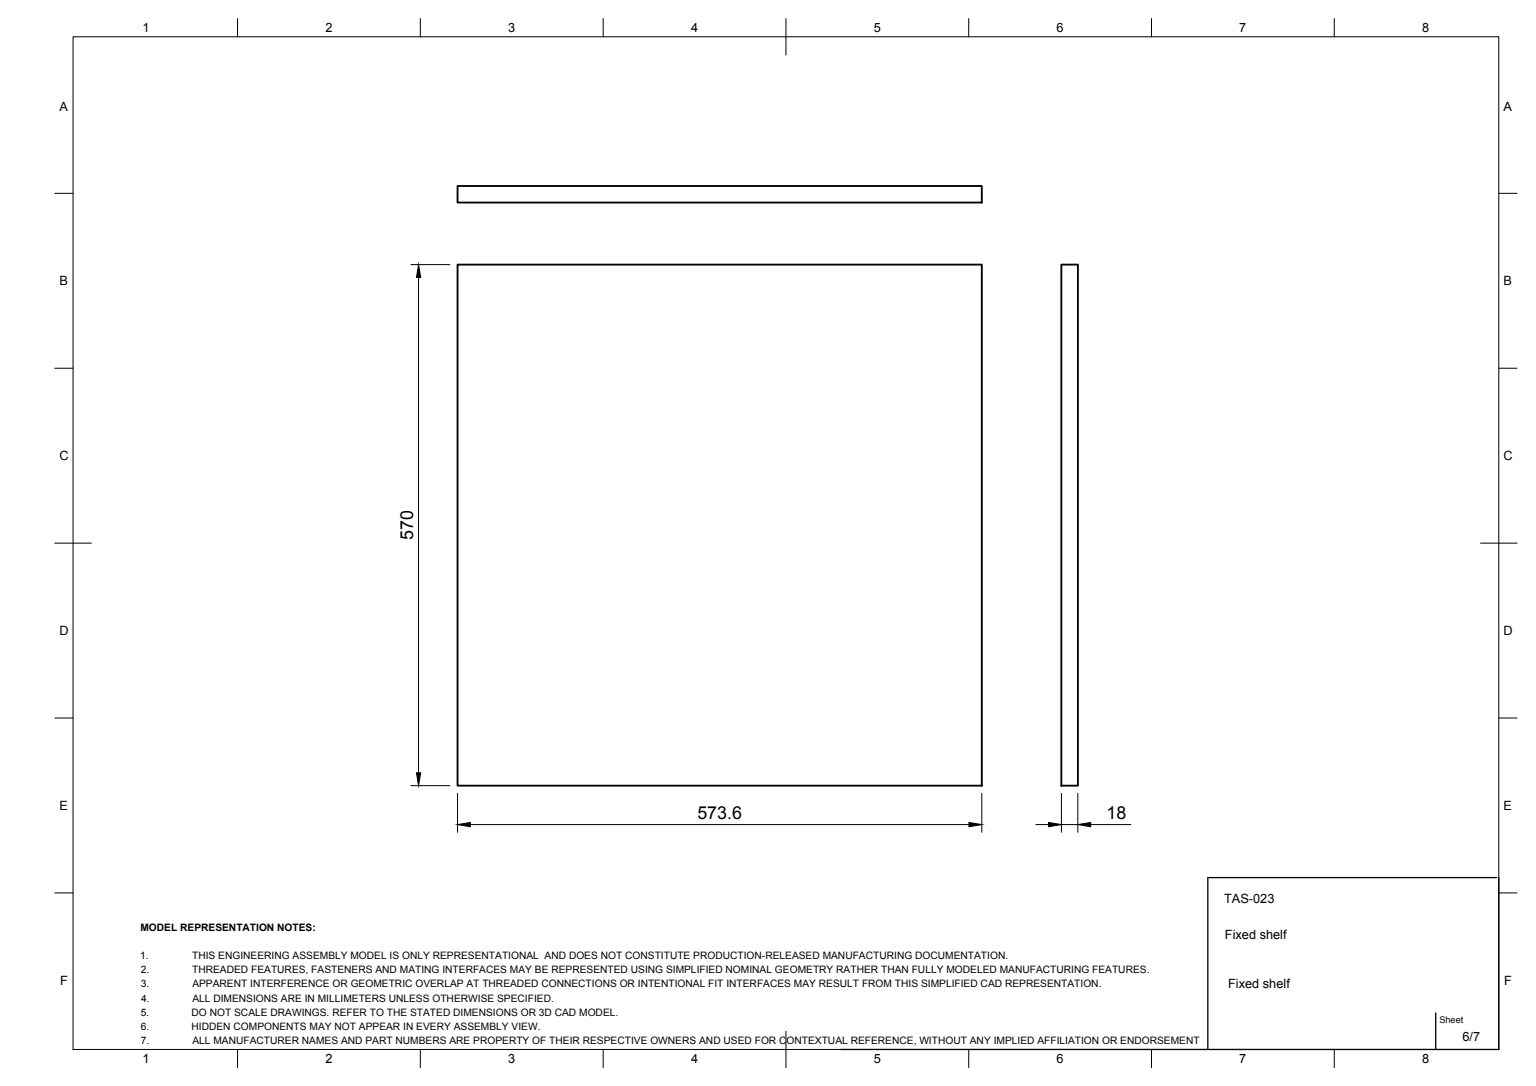
ISO-10303-21;
HEADER;
/* Generated by software containing ST-Developer
 * from STEP Tools, Inc. (www.steptools.com) 
 */

FILE_DESCRIPTION(
/* description */ (''),
/* implementation_level */ '2;1');

FILE_NAME(
/* name */ 'Fixed shelf.step',
/* time_stamp */ '2026-11-15T17:51:54-08:00',
/* author */ (''),
/* organization */ (''),
/* preprocessor_version */ 'ST-DEVELOPER v20.2',
/* originating_system */ 'Autodesk Translation Framework v15.17.0.0',
/* authorisation */ '');

FILE_SCHEMA (('AUTOMOTIVE_DESIGN { 1 0 10303 214 3 1 1 }'));
ENDSEC;

DATA;
#10=MECHANICAL_DESIGN_GEOMETRIC_PRESENTATION_REPRESENTATION('',(#120),#2860);
#110=SHAPE_REPRESENTATION_RELATIONSHIP('SRR','None',#2905,#115);
#115=ADVANCED_BREP_SHAPE_REPRESENTATION('',(#125),#2858);
#120=STYLED_ITEM('',(#2939),#125);
#125=MANIFOLD_SOLID_BREP('Body1',#1717);
#205=PLANE('',#1866);
#206=PLANE('',#1867);
#207=PLANE('',#1868);
#208=PLANE('',#1869);
#209=PLANE('',#1870);
#210=PLANE('',#1871);
#291=FACE_OUTER_BOUND('',#382,.T.);
#292=FACE_OUTER_BOUND('',#383,.T.);
#293=FACE_OUTER_BOUND('',#384,.T.);
#294=FACE_OUTER_BOUND('',#385,.T.);
#295=FACE_OUTER_BOUND('',#386,.T.);
#296=FACE_OUTER_BOUND('',#387,.T.);
#382=EDGE_LOOP('',(#1592,#1593,#1594,#1595));
#383=EDGE_LOOP('',(#1596,#1597,#1598,#1599));
#384=EDGE_LOOP('',(#1600,#1601,#1602,#1603));
#385=EDGE_LOOP('',(#1604,#1605,#1606,#1607));
#386=EDGE_LOOP('',(#1608,#1609,#1610,#1611));
#387=EDGE_LOOP('',(#1612,#1613,#1614,#1615));
#587=LINE('',#2791,#796);
#588=LINE('',#2793,#797);
#589=LINE('',#2795,#798);
#590=LINE('',#2796,#799);
#591=LINE('',#2799,#800);
#592=LINE('',#2801,#801);
#593=LINE('',#2802,#802);
#594=LINE('',#2805,#803);
#595=LINE('',#2807,#804);
#596=LINE('',#2808,#805);
#597=LINE('',#2810,#806);
#598=LINE('',#2811,#807);
#796=VECTOR('',#2282,1.);
#797=VECTOR('',#2283,1.);
#798=VECTOR('',#2284,1.);
#799=VECTOR('',#2285,1.);
#800=VECTOR('',#2288,1.);
#801=VECTOR('',#2289,1.);
#802=VECTOR('',#2290,1.);
#803=VECTOR('',#2293,1.);
#804=VECTOR('',#2294,1.);
#805=VECTOR('',#2295,1.);
#806=VECTOR('',#2298,1.);
#807=VECTOR('',#2299,1.);
#955=VERTEX_POINT('',#2789);
#956=VERTEX_POINT('',#2790);
#957=VERTEX_POINT('',#2792);
#958=VERTEX_POINT('',#2794);
#959=VERTEX_POINT('',#2798);
#960=VERTEX_POINT('',#2800);
#961=VERTEX_POINT('',#2804);
#962=VERTEX_POINT('',#2806);
#1169=EDGE_CURVE('',#955,#956,#587,.T.);
#1170=EDGE_CURVE('',#956,#957,#588,.T.);
#1171=EDGE_CURVE('',#958,#957,#589,.T.);
#1172=EDGE_CURVE('',#955,#958,#590,.T.);
#1173=EDGE_CURVE('',#959,#955,#591,.T.);
#1174=EDGE_CURVE('',#960,#958,#592,.T.);
#1175=EDGE_CURVE('',#959,#960,#593,.T.);
#1176=EDGE_CURVE('',#961,#959,#594,.T.);
#1177=EDGE_CURVE('',#962,#960,#595,.T.);
#1178=EDGE_CURVE('',#961,#962,#596,.T.);
#1179=EDGE_CURVE('',#956,#961,#597,.T.);
#1180=EDGE_CURVE('',#957,#962,#598,.T.);
#1592=ORIENTED_EDGE('',*,*,#1169,.T.);
#1593=ORIENTED_EDGE('',*,*,#1170,.T.);
#1594=ORIENTED_EDGE('',*,*,#1171,.F.);
#1595=ORIENTED_EDGE('',*,*,#1172,.F.);
#1596=ORIENTED_EDGE('',*,*,#1173,.T.);
#1597=ORIENTED_EDGE('',*,*,#1172,.T.);
#1598=ORIENTED_EDGE('',*,*,#1174,.F.);
#1599=ORIENTED_EDGE('',*,*,#1175,.F.);
#1600=ORIENTED_EDGE('',*,*,#1176,.T.);
#1601=ORIENTED_EDGE('',*,*,#1175,.T.);
#1602=ORIENTED_EDGE('',*,*,#1177,.F.);
#1603=ORIENTED_EDGE('',*,*,#1178,.F.);
#1604=ORIENTED_EDGE('',*,*,#1179,.T.);
#1605=ORIENTED_EDGE('',*,*,#1178,.T.);
#1606=ORIENTED_EDGE('',*,*,#1180,.F.);
#1607=ORIENTED_EDGE('',*,*,#1170,.F.);
#1608=ORIENTED_EDGE('',*,*,#1180,.T.);
#1609=ORIENTED_EDGE('',*,*,#1177,.T.);
#1610=ORIENTED_EDGE('',*,*,#1174,.T.);
#1611=ORIENTED_EDGE('',*,*,#1171,.T.);
#1612=ORIENTED_EDGE('',*,*,#1179,.F.);
#1613=ORIENTED_EDGE('',*,*,#1169,.F.);
#1614=ORIENTED_EDGE('',*,*,#1173,.F.);
#1615=ORIENTED_EDGE('',*,*,#1176,.F.);
#1705=ADVANCED_FACE('',(#291),#205,.T.);
#1706=ADVANCED_FACE('',(#292),#206,.T.);
#1707=ADVANCED_FACE('',(#293),#207,.T.);
#1708=ADVANCED_FACE('',(#294),#208,.T.);
#1709=ADVANCED_FACE('',(#295),#209,.T.);
#1710=ADVANCED_FACE('',(#296),#210,.F.);
#1717=CLOSED_SHELL('',(#1705,#1706,#1707,#1708,#1709,#1710));
#1865=AXIS2_PLACEMENT_3D('',#2787,#2278,#2279);
#1866=AXIS2_PLACEMENT_3D('',#2788,#2280,#2281);
#1867=AXIS2_PLACEMENT_3D('',#2797,#2286,#2287);
#1868=AXIS2_PLACEMENT_3D('',#2803,#2291,#2292);
#1869=AXIS2_PLACEMENT_3D('',#2809,#2296,#2297);
#1870=AXIS2_PLACEMENT_3D('',#2812,#2300,#2301);
#1871=AXIS2_PLACEMENT_3D('',#2813,#2302,#2303);
#2278=DIRECTION('axis',(0.,0.,1.));
#2279=DIRECTION('refdir',(1.,0.,0.));
#2280=DIRECTION('center_axis',(0.,1.,0.));
#2281=DIRECTION('ref_axis',(-1.,0.,0.));
#2282=DIRECTION('',(-1.,0.,0.));
#2283=DIRECTION('',(0.,0.,1.));
#2284=DIRECTION('',(-1.,0.,0.));
#2285=DIRECTION('',(0.,0.,1.));
#2286=DIRECTION('center_axis',(1.,0.,0.));
#2287=DIRECTION('ref_axis',(0.,1.,0.));
#2288=DIRECTION('',(0.,1.,0.));
#2289=DIRECTION('',(0.,1.,0.));
#2290=DIRECTION('',(0.,0.,1.));
#2291=DIRECTION('center_axis',(0.,-1.,0.));
#2292=DIRECTION('ref_axis',(1.,0.,0.));
#2293=DIRECTION('',(1.,0.,0.));
#2294=DIRECTION('',(1.,0.,0.));
#2295=DIRECTION('',(0.,0.,1.));
#2296=DIRECTION('center_axis',(-1.,0.,0.));
#2297=DIRECTION('ref_axis',(0.,-1.,0.));
#2298=DIRECTION('',(0.,-1.,0.));
#2299=DIRECTION('',(0.,-1.,0.));
#2300=DIRECTION('center_axis',(0.,0.,1.));
#2301=DIRECTION('ref_axis',(1.,0.,0.));
#2302=DIRECTION('center_axis',(0.,0.,1.));
#2303=DIRECTION('ref_axis',(1.,0.,0.));
#2787=CARTESIAN_POINT('',(0.,0.,0.));
#2788=CARTESIAN_POINT('Origin',(57.36,57.6,0.));
#2789=CARTESIAN_POINT('',(57.36,57.6,0.));
#2790=CARTESIAN_POINT('',(0.,57.6,0.));
#2791=CARTESIAN_POINT('',(57.36,57.6,0.));
#2792=CARTESIAN_POINT('',(0.,57.6,1.8));
#2793=CARTESIAN_POINT('',(0.,57.6,0.));
#2794=CARTESIAN_POINT('',(57.36,57.6,1.8));
#2795=CARTESIAN_POINT('',(57.36,57.6,1.8));
#2796=CARTESIAN_POINT('',(57.36,57.6,0.));
#2797=CARTESIAN_POINT('Origin',(57.36,0.6,0.));
#2798=CARTESIAN_POINT('',(57.36,0.6,0.));
#2799=CARTESIAN_POINT('',(57.36,0.6,0.));
#2800=CARTESIAN_POINT('',(57.36,0.600000000000001,1.8));
#2801=CARTESIAN_POINT('',(57.36,0.6,1.8));
#2802=CARTESIAN_POINT('',(57.36,0.6,0.));
#2803=CARTESIAN_POINT('Origin',(0.,0.6,0.));
#2804=CARTESIAN_POINT('',(0.,0.600000000000001,0.));
#2805=CARTESIAN_POINT('',(0.,0.6,0.));
#2806=CARTESIAN_POINT('',(0.,0.600000000000001,1.8));
#2807=CARTESIAN_POINT('',(0.,0.6,1.8));
#2808=CARTESIAN_POINT('',(0.,0.600000000000001,0.));
#2809=CARTESIAN_POINT('Origin',(0.,57.6,0.));
#2810=CARTESIAN_POINT('',(0.,57.6,0.));
#2811=CARTESIAN_POINT('',(0.,57.6,1.8));
#2812=CARTESIAN_POINT('Origin',(28.68,29.1,1.8));
#2813=CARTESIAN_POINT('Origin',(28.68,29.1,0.));
#2851=UNCERTAINTY_MEASURE_WITH_UNIT(LENGTH_MEASURE(0.001),#2861,
'DISTANCE_ACCURACY_VALUE',
'Maximum model space distance between geometric entities at asserted c
onnectivities');
#2853=UNCERTAINTY_MEASURE_WITH_UNIT(LENGTH_MEASURE(0.001),#2861,
'DISTANCE_ACCURACY_VALUE',
'Maximum model space distance between geometric entities at asserted c
onnectivities');
#2858=(
GEOMETRIC_REPRESENTATION_CONTEXT(3)
GLOBAL_UNCERTAINTY_ASSIGNED_CONTEXT((#2851))
GLOBAL_UNIT_ASSIGNED_CONTEXT((#2861,#2863,#2864))
REPRESENTATION_CONTEXT('','3D')
);
#2860=(
GEOMETRIC_REPRESENTATION_CONTEXT(3)
GLOBAL_UNCERTAINTY_ASSIGNED_CONTEXT((#2853))
GLOBAL_UNIT_ASSIGNED_CONTEXT((#2861,#2863,#2864))
REPRESENTATION_CONTEXT('','3D')
);
#2861=(
LENGTH_UNIT()
NAMED_UNIT(*)
SI_UNIT(.CENTI.,.METRE.)
);
#2863=(
NAMED_UNIT(*)
PLANE_ANGLE_UNIT()
SI_UNIT($,.RADIAN.)
);
#2864=(
NAMED_UNIT(*)
SI_UNIT($,.STERADIAN.)
SOLID_ANGLE_UNIT()
);
#2869=SHAPE_DEFINITION_REPRESENTATION(#2875,#2905);
#2875=PRODUCT_DEFINITION_SHAPE('',$,#2912);
#2905=SHAPE_REPRESENTATION('',(#1865),#2858);
#2907=PRODUCT_DEFINITION_CONTEXT('part definition',#2927,'design');
#2912=PRODUCT_DEFINITION('Fixed shelf','Fixed shelf',#2918,#2907);
#2918=PRODUCT_DEFINITION_FORMATION('',$,#2933);
#2927=APPLICATION_CONTEXT(
'Core Data for Automotive Mechanical Design Process');
#2928=PRODUCT_CONTEXT('part definition',#2927,'mechanical');
#2933=PRODUCT('Fixed shelf','Fixed shelf',$,(#2928));
#2939=PRESENTATION_STYLE_ASSIGNMENT((#2945));
#2945=SURFACE_STYLE_USAGE(.BOTH.,#2951);
#2951=SURFACE_SIDE_STYLE('',(#2957));
#2957=SURFACE_STYLE_FILL_AREA(#2963);
#2963=FILL_AREA_STYLE('Fixed shelf finish',(#2969));
#2969=FILL_AREA_STYLE_COLOUR('Fixed shelf finish',#2975);
#2975=COLOUR_RGB('Fixed shelf finish',0.274509803921569,0.6,0.8);
ENDSEC;
END-ISO-10303-21;
